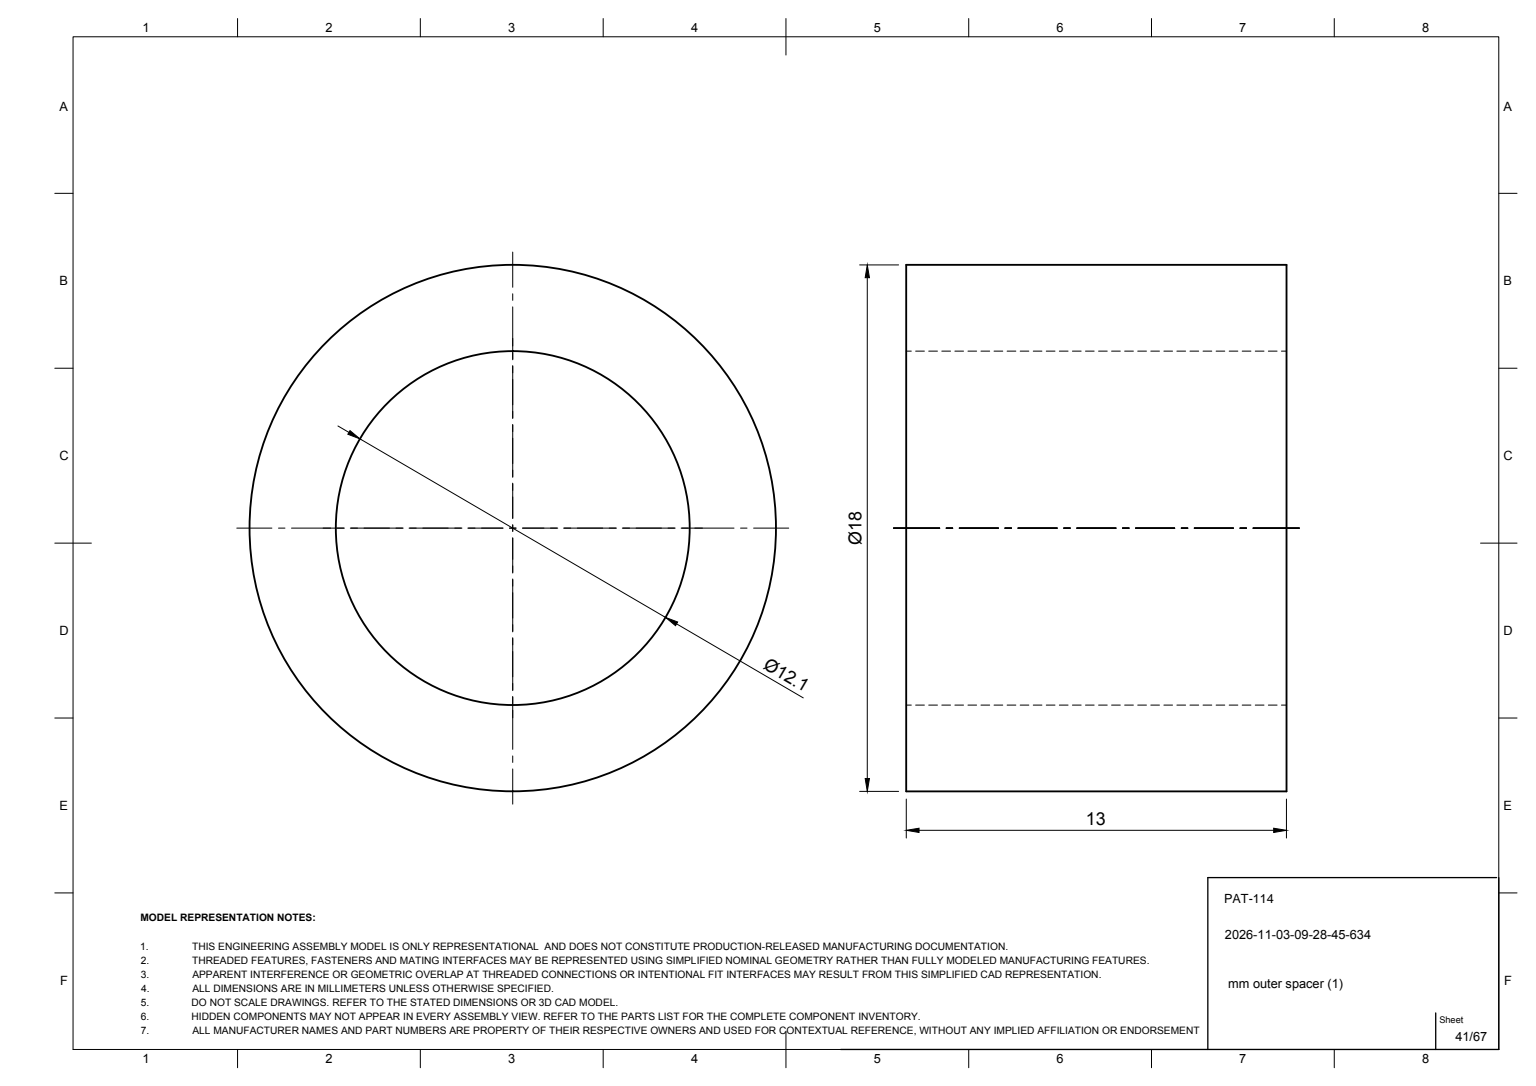
ISO-10303-21;
HEADER;
/* Generated by software containing ST-Developer
 * from STEP Tools, Inc. (www.steptools.com) 
 */

FILE_DESCRIPTION(
/* description */ ('Two-stage gear reducer in split housing'),
/* implementation_level */ '2;1');

FILE_NAME(
/* name */ 'mm outer spacer (1).step',
/* time_stamp */ '2026-10-28T03:22:31-07:00',
/* author */ (''),
/* organization */ (''),
/* preprocessor_version */ 'ST-DEVELOPER v20.2',
/* originating_system */ 'Autodesk Translation Framework v15.17.0.0',
/* authorisation */ '');

FILE_SCHEMA (('AUTOMOTIVE_DESIGN { 1 0 10303 214 3 1 1 }'));
ENDSEC;

DATA;
#10=MECHANICAL_DESIGN_GEOMETRIC_PRESENTATION_REPRESENTATION('',(#1281),#73366);
#1154=SHAPE_REPRESENTATION_RELATIONSHIP('SRR','None',#73644,#1210);
#1210=ADVANCED_BREP_SHAPE_REPRESENTATION('',(#1350),#73340);
#1281=STYLED_ITEM('',(#73974),#1350);
#1350=MANIFOLD_SOLID_BREP('Body1',#16171);
#1549=FACE_BOUND('',#3533,.T.);
#1550=FACE_BOUND('',#3535,.T.);
#1816=PLANE('',#17824);
#1817=PLANE('',#17825);
#2442=FACE_OUTER_BOUND('',#3530,.T.);
#2443=FACE_OUTER_BOUND('',#3531,.T.);
#2444=FACE_OUTER_BOUND('',#3532,.T.);
#2445=FACE_OUTER_BOUND('',#3534,.T.);
#3530=EDGE_LOOP('',(#12395,#12396,#12397,#12398));
#3531=EDGE_LOOP('',(#12399,#12400,#12401,#12402));
#3532=EDGE_LOOP('',(#12403));
#3533=EDGE_LOOP('',(#12404));
#3534=EDGE_LOOP('',(#12405));
#3535=EDGE_LOOP('',(#12406));
#4502=LINE('',#25651,#5526);
#4503=LINE('',#25657,#5527);
#5526=VECTOR('',#20920,0.605);
#5527=VECTOR('',#20927,0.9);
#6562=CIRCLE('',#17819,0.605);
#6563=CIRCLE('',#17820,0.605);
#6564=CIRCLE('',#17822,0.9);
#6565=CIRCLE('',#17823,0.9);
#7469=VERTEX_POINT('',#25648);
#7470=VERTEX_POINT('',#25650);
#7471=VERTEX_POINT('',#25654);
#7472=VERTEX_POINT('',#25656);
#9251=EDGE_CURVE('',#7469,#7469,#6562,.T.);
#9252=EDGE_CURVE('',#7469,#7470,#4502,.T.);
#9253=EDGE_CURVE('',#7470,#7470,#6563,.T.);
#9254=EDGE_CURVE('',#7471,#7471,#6564,.T.);
#9255=EDGE_CURVE('',#7471,#7472,#4503,.T.);
#9256=EDGE_CURVE('',#7472,#7472,#6565,.T.);
#12395=ORIENTED_EDGE('',*,*,#9251,.F.);
#12396=ORIENTED_EDGE('',*,*,#9252,.T.);
#12397=ORIENTED_EDGE('',*,*,#9253,.T.);
#12398=ORIENTED_EDGE('',*,*,#9252,.F.);
#12399=ORIENTED_EDGE('',*,*,#9254,.F.);
#12400=ORIENTED_EDGE('',*,*,#9255,.T.);
#12401=ORIENTED_EDGE('',*,*,#9256,.T.);
#12402=ORIENTED_EDGE('',*,*,#9255,.F.);
#12403=ORIENTED_EDGE('',*,*,#9254,.T.);
#12404=ORIENTED_EDGE('',*,*,#9251,.T.);
#12405=ORIENTED_EDGE('',*,*,#9256,.F.);
#12406=ORIENTED_EDGE('',*,*,#9253,.F.);
#15084=CYLINDRICAL_SURFACE('',#17818,0.605);
#15085=CYLINDRICAL_SURFACE('',#17821,0.9);
#15649=ADVANCED_FACE('',(#2442),#15084,.F.);
#15650=ADVANCED_FACE('',(#2443),#15085,.T.);
#15651=ADVANCED_FACE('',(#2444,#1549),#1816,.T.);
#15652=ADVANCED_FACE('',(#2445,#1550),#1817,.F.);
#16171=CLOSED_SHELL('',(#15649,#15650,#15651,#15652));
#17817=AXIS2_PLACEMENT_3D('',#25646,#20914,#20915);
#17818=AXIS2_PLACEMENT_3D('',#25647,#20916,#20917);
#17819=AXIS2_PLACEMENT_3D('',#25649,#20918,#20919);
#17820=AXIS2_PLACEMENT_3D('',#25652,#20921,#20922);
#17821=AXIS2_PLACEMENT_3D('',#25653,#20923,#20924);
#17822=AXIS2_PLACEMENT_3D('',#25655,#20925,#20926);
#17823=AXIS2_PLACEMENT_3D('',#25658,#20928,#20929);
#17824=AXIS2_PLACEMENT_3D('',#25659,#20930,#20931);
#17825=AXIS2_PLACEMENT_3D('',#25660,#20932,#20933);
#20914=DIRECTION('axis',(0.,0.,1.));
#20915=DIRECTION('refdir',(1.,0.,0.));
#20916=DIRECTION('center_axis',(0.,1.,0.));
#20917=DIRECTION('ref_axis',(1.,0.,0.));
#20918=DIRECTION('center_axis',(0.,-1.,0.));
#20919=DIRECTION('ref_axis',(1.,0.,0.));
#20920=DIRECTION('',(0.,-1.,0.));
#20921=DIRECTION('center_axis',(0.,-1.,0.));
#20922=DIRECTION('ref_axis',(1.,0.,0.));
#20923=DIRECTION('center_axis',(0.,1.,0.));
#20924=DIRECTION('ref_axis',(1.,0.,0.));
#20925=DIRECTION('center_axis',(0.,1.,0.));
#20926=DIRECTION('ref_axis',(1.,0.,0.));
#20927=DIRECTION('',(0.,-1.,0.));
#20928=DIRECTION('center_axis',(0.,1.,0.));
#20929=DIRECTION('ref_axis',(1.,0.,0.));
#20930=DIRECTION('center_axis',(0.,1.,0.));
#20931=DIRECTION('ref_axis',(1.,0.,0.));
#20932=DIRECTION('center_axis',(0.,1.,0.));
#20933=DIRECTION('ref_axis',(1.,0.,0.));
#25646=CARTESIAN_POINT('',(0.,0.,0.));
#25647=CARTESIAN_POINT('Origin',(0.,6.5,10.));
#25648=CARTESIAN_POINT('',(-0.605,7.8,10.));
#25649=CARTESIAN_POINT('Origin',(0.,7.8,10.));
#25650=CARTESIAN_POINT('',(-0.605,6.5,10.));
#25651=CARTESIAN_POINT('',(-0.605,6.5,10.));
#25652=CARTESIAN_POINT('Origin',(0.,6.5,10.));
#25653=CARTESIAN_POINT('Origin',(0.,6.5,10.));
#25654=CARTESIAN_POINT('',(-0.9,7.8,10.));
#25655=CARTESIAN_POINT('Origin',(0.,7.8,10.));
#25656=CARTESIAN_POINT('',(-0.9,6.5,10.));
#25657=CARTESIAN_POINT('',(-0.9,6.5,10.));
#25658=CARTESIAN_POINT('Origin',(0.,6.5,10.));
#25659=CARTESIAN_POINT('Origin',(0.,7.8,10.));
#25660=CARTESIAN_POINT('Origin',(0.,6.5,10.));
#73276=UNCERTAINTY_MEASURE_WITH_UNIT(LENGTH_MEASURE(0.001),#73367,
'DISTANCE_ACCURACY_VALUE',
'Maximum model space distance between geometric entities at asserted c
onnectivities');
#73302=UNCERTAINTY_MEASURE_WITH_UNIT(LENGTH_MEASURE(0.001),#73367,
'DISTANCE_ACCURACY_VALUE',
'Maximum model space distance between geometric entities at asserted c
onnectivities');
#73340=(
GEOMETRIC_REPRESENTATION_CONTEXT(3)
GLOBAL_UNCERTAINTY_ASSIGNED_CONTEXT((#73276))
GLOBAL_UNIT_ASSIGNED_CONTEXT((#73367,#73369,#73370))
REPRESENTATION_CONTEXT('','3D')
);
#73366=(
GEOMETRIC_REPRESENTATION_CONTEXT(3)
GLOBAL_UNCERTAINTY_ASSIGNED_CONTEXT((#73302))
GLOBAL_UNIT_ASSIGNED_CONTEXT((#73367,#73369,#73370))
REPRESENTATION_CONTEXT('','3D')
);
#73367=(
LENGTH_UNIT()
NAMED_UNIT(*)
SI_UNIT(.CENTI.,.METRE.)
);
#73369=(
NAMED_UNIT(*)
PLANE_ANGLE_UNIT()
SI_UNIT($,.RADIAN.)
);
#73370=(
NAMED_UNIT(*)
SI_UNIT($,.STERADIAN.)
SOLID_ANGLE_UNIT()
);
#73408=SHAPE_DEFINITION_REPRESENTATION(#73541,#73644);
#73541=PRODUCT_DEFINITION_SHAPE('',$,#73708);
#73644=SHAPE_REPRESENTATION('',(#17817),#73340);
#73670=PRODUCT_DEFINITION_CONTEXT('part definition',#73861,'design');
#73708=PRODUCT_DEFINITION('mm outer spacer (1)','mm outer spacer (1)',#73771,
#73670);
#73771=PRODUCT_DEFINITION_FORMATION('',$,#73900);
#73861=APPLICATION_CONTEXT(
'Core Data for Automotive Mechanical Design Process');
#73862=PRODUCT_CONTEXT('part definition',#73861,'mechanical');
#73900=PRODUCT('mm outer spacer (1)','mm outer spacer (1)',
'mm outer spacer (1)',(#73862));
#73968=COLOUR_RGB('Light Blue',0.38,0.62,0.78);
#73969=FILL_AREA_STYLE_COLOUR('',#73968);
#73970=FILL_AREA_STYLE('',(#73969));
#73971=SURFACE_STYLE_FILL_AREA(#73970);
#73972=SURFACE_SIDE_STYLE('',(#73971));
#73973=SURFACE_STYLE_USAGE(.BOTH.,#73972);
#73974=PRESENTATION_STYLE_ASSIGNMENT((#73973));
ENDSEC;
END-ISO-10303-21;
